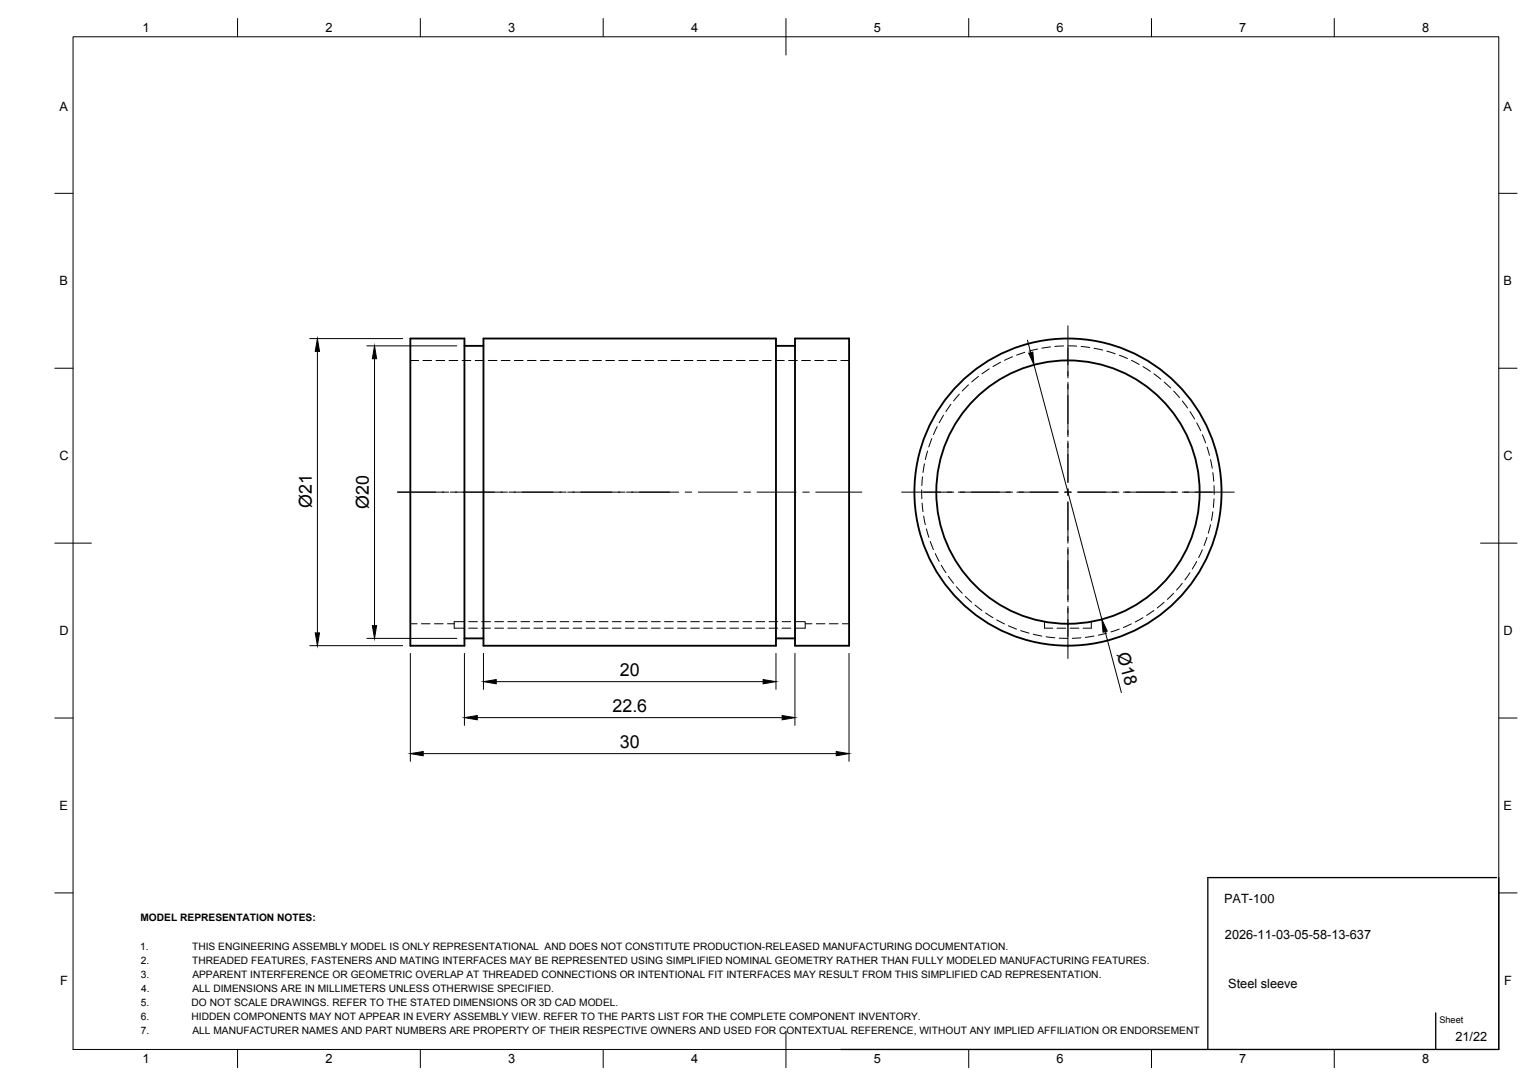
ISO-10303-21;
HEADER;
/* Generated by software containing ST-Developer
 * from STEP Tools, Inc. (www.steptools.com) 
 */

FILE_DESCRIPTION(
/* description */ (''),
/* implementation_level */ '2;1');

FILE_NAME(
/* name */ 'Steel sleeve.step',
/* time_stamp */ '2026-10-29T16:43:51-07:00',
/* author */ (''),
/* organization */ (''),
/* preprocessor_version */ 'ST-DEVELOPER v20.2',
/* originating_system */ 'Autodesk Translation Framework v15.17.0.0',
/* authorisation */ '');

FILE_SCHEMA (('AUTOMOTIVE_DESIGN { 1 0 10303 214 3 1 1 }'));
ENDSEC;

DATA;
#10=MECHANICAL_DESIGN_GEOMETRIC_PRESENTATION_REPRESENTATION('',(#380),#10292);
#334=SHAPE_REPRESENTATION_RELATIONSHIP('SRR','None',#10432,#357);
#357=ADVANCED_BREP_SHAPE_REPRESENTATION('',(#401),#10284);
#380=STYLED_ITEM('',(#10642),#401);
#401=MANIFOLD_SOLID_BREP('Body1',#5024);
#501=FACE_BOUND('',#1291,.T.);
#502=FACE_BOUND('',#1294,.T.);
#503=FACE_BOUND('',#1297,.T.);
#504=FACE_BOUND('',#1300,.T.);
#505=FACE_BOUND('',#1303,.T.);
#506=FACE_BOUND('',#1306,.T.);
#507=FACE_BOUND('',#1308,.T.);
#650=PLANE('',#5633);
#651=PLANE('',#5635);
#652=PLANE('',#5636);
#653=PLANE('',#5638);
#654=PLANE('',#5639);
#655=PLANE('',#5640);
#656=PLANE('',#5645);
#657=PLANE('',#5649);
#658=PLANE('',#5653);
#659=PLANE('',#5657);
#660=PLANE('',#5661);
#902=FACE_OUTER_BOUND('',#1285,.T.);
#903=FACE_OUTER_BOUND('',#1286,.T.);
#904=FACE_OUTER_BOUND('',#1287,.T.);
#905=FACE_OUTER_BOUND('',#1288,.T.);
#906=FACE_OUTER_BOUND('',#1289,.T.);
#907=FACE_OUTER_BOUND('',#1290,.T.);
#908=FACE_OUTER_BOUND('',#1292,.T.);
#909=FACE_OUTER_BOUND('',#1293,.T.);
#910=FACE_OUTER_BOUND('',#1295,.T.);
#911=FACE_OUTER_BOUND('',#1296,.T.);
#912=FACE_OUTER_BOUND('',#1298,.T.);
#913=FACE_OUTER_BOUND('',#1299,.T.);
#914=FACE_OUTER_BOUND('',#1301,.T.);
#915=FACE_OUTER_BOUND('',#1302,.T.);
#916=FACE_OUTER_BOUND('',#1304,.T.);
#917=FACE_OUTER_BOUND('',#1305,.T.);
#918=FACE_OUTER_BOUND('',#1307,.T.);
#1285=EDGE_LOOP('',(#4265,#4266,#4267,#4268));
#1286=EDGE_LOOP('',(#4269,#4270,#4271,#4272));
#1287=EDGE_LOOP('',(#4273,#4274,#4275,#4276));
#1288=EDGE_LOOP('',(#4277,#4278,#4279,#4280));
#1289=EDGE_LOOP('',(#4281,#4282,#4283,#4284));
#1290=EDGE_LOOP('',(#4285));
#1291=EDGE_LOOP('',(#4286));
#1292=EDGE_LOOP('',(#4287,#4288,#4289,#4290));
#1293=EDGE_LOOP('',(#4291));
#1294=EDGE_LOOP('',(#4292));
#1295=EDGE_LOOP('',(#4293,#4294,#4295,#4296));
#1296=EDGE_LOOP('',(#4297));
#1297=EDGE_LOOP('',(#4298));
#1298=EDGE_LOOP('',(#4299,#4300,#4301,#4302));
#1299=EDGE_LOOP('',(#4303));
#1300=EDGE_LOOP('',(#4304));
#1301=EDGE_LOOP('',(#4305,#4306,#4307,#4308));
#1302=EDGE_LOOP('',(#4309));
#1303=EDGE_LOOP('',(#4310));
#1304=EDGE_LOOP('',(#4311,#4312,#4313,#4314));
#1305=EDGE_LOOP('',(#4315));
#1306=EDGE_LOOP('',(#4316));
#1307=EDGE_LOOP('',(#4317,#4318,#4319,#4320));
#1308=EDGE_LOOP('',(#4321,#4322,#4323,#4324));
#1683=LINE('',#9771,#2075);
#1684=LINE('',#9773,#2076);
#1685=LINE('',#9774,#2077);
#1686=LINE('',#9777,#2078);
#1687=LINE('',#9779,#2079);
#1688=LINE('',#9780,#2080);
#1689=LINE('',#9785,#2081);
#1690=LINE('',#9786,#2082);
#1691=LINE('',#9788,#2083);
#1692=LINE('',#9789,#2084);
#1693=LINE('',#9799,#2085);
#1694=LINE('',#9806,#2086);
#1695=LINE('',#9813,#2087);
#1696=LINE('',#9820,#2088);
#1697=LINE('',#9827,#2089);
#1698=LINE('',#9832,#2090);
#2075=VECTOR('',#6828,1.);
#2076=VECTOR('',#6829,1.);
#2077=VECTOR('',#6830,1.);
#2078=VECTOR('',#6833,1.);
#2079=VECTOR('',#6834,1.);
#2080=VECTOR('',#6835,1.);
#2081=VECTOR('',#6840,1.);
#2082=VECTOR('',#6841,1.);
#2083=VECTOR('',#6844,1.);
#2084=VECTOR('',#6845,1.);
#2085=VECTOR('',#6858,1.05);
#2086=VECTOR('',#6867,1.);
#2087=VECTOR('',#6876,1.05);
#2088=VECTOR('',#6885,1.);
#2089=VECTOR('',#6894,1.05);
#2090=VECTOR('',#6901,0.9);
#2328=CIRCLE('',#5634,0.9);
#2329=CIRCLE('',#5637,0.9);
#2330=CIRCLE('',#5641,1.05);
#2331=CIRCLE('',#5642,0.9);
#2332=CIRCLE('',#5644,1.05);
#2333=CIRCLE('',#5646,1.);
#2334=CIRCLE('',#5648,1.);
#2335=CIRCLE('',#5650,1.05);
#2336=CIRCLE('',#5652,1.05);
#2337=CIRCLE('',#5654,1.);
#2338=CIRCLE('',#5656,1.);
#2339=CIRCLE('',#5658,1.05);
#2340=CIRCLE('',#5660,1.05);
#2341=CIRCLE('',#5662,0.9);
#2675=VERTEX_POINT('',#9767);
#2676=VERTEX_POINT('',#9768);
#2677=VERTEX_POINT('',#9770);
#2678=VERTEX_POINT('',#9772);
#2679=VERTEX_POINT('',#9776);
#2680=VERTEX_POINT('',#9778);
#2681=VERTEX_POINT('',#9782);
#2682=VERTEX_POINT('',#9784);
#2683=VERTEX_POINT('',#9792);
#2684=VERTEX_POINT('',#9794);
#2685=VERTEX_POINT('',#9797);
#2686=VERTEX_POINT('',#9801);
#2687=VERTEX_POINT('',#9804);
#2688=VERTEX_POINT('',#9808);
#2689=VERTEX_POINT('',#9811);
#2690=VERTEX_POINT('',#9815);
#2691=VERTEX_POINT('',#9818);
#2692=VERTEX_POINT('',#9822);
#2693=VERTEX_POINT('',#9825);
#2694=VERTEX_POINT('',#9829);
#3223=EDGE_CURVE('',#2675,#2676,#2328,.T.);
#3224=EDGE_CURVE('',#2677,#2675,#1683,.T.);
#3225=EDGE_CURVE('',#2678,#2677,#1684,.T.);
#3226=EDGE_CURVE('',#2676,#2678,#1685,.T.);
#3227=EDGE_CURVE('',#2676,#2679,#1686,.T.);
#3228=EDGE_CURVE('',#2680,#2678,#1687,.T.);
#3229=EDGE_CURVE('',#2680,#2679,#1688,.T.);
#3230=EDGE_CURVE('',#2679,#2681,#2329,.T.);
#3231=EDGE_CURVE('',#2682,#2680,#1689,.T.);
#3232=EDGE_CURVE('',#2681,#2682,#1690,.T.);
#3233=EDGE_CURVE('',#2681,#2675,#1691,.T.);
#3234=EDGE_CURVE('',#2682,#2677,#1692,.T.);
#3235=EDGE_CURVE('',#2683,#2683,#2330,.T.);
#3236=EDGE_CURVE('',#2684,#2684,#2331,.T.);
#3237=EDGE_CURVE('',#2685,#2685,#2332,.T.);
#3238=EDGE_CURVE('',#2685,#2683,#1693,.T.);
#3239=EDGE_CURVE('',#2686,#2686,#2333,.T.);
#3240=EDGE_CURVE('',#2687,#2687,#2334,.T.);
#3241=EDGE_CURVE('',#2687,#2686,#1694,.T.);
#3242=EDGE_CURVE('',#2688,#2688,#2335,.T.);
#3243=EDGE_CURVE('',#2689,#2689,#2336,.T.);
#3244=EDGE_CURVE('',#2689,#2688,#1695,.T.);
#3245=EDGE_CURVE('',#2690,#2690,#2337,.T.);
#3246=EDGE_CURVE('',#2691,#2691,#2338,.T.);
#3247=EDGE_CURVE('',#2691,#2690,#1696,.T.);
#3248=EDGE_CURVE('',#2692,#2692,#2339,.T.);
#3249=EDGE_CURVE('',#2693,#2693,#2340,.T.);
#3250=EDGE_CURVE('',#2693,#2692,#1697,.T.);
#3251=EDGE_CURVE('',#2694,#2694,#2341,.T.);
#3252=EDGE_CURVE('',#2694,#2684,#1698,.T.);
#4265=ORIENTED_EDGE('',*,*,#3223,.F.);
#4266=ORIENTED_EDGE('',*,*,#3224,.F.);
#4267=ORIENTED_EDGE('',*,*,#3225,.F.);
#4268=ORIENTED_EDGE('',*,*,#3226,.F.);
#4269=ORIENTED_EDGE('',*,*,#3227,.F.);
#4270=ORIENTED_EDGE('',*,*,#3226,.T.);
#4271=ORIENTED_EDGE('',*,*,#3228,.F.);
#4272=ORIENTED_EDGE('',*,*,#3229,.T.);
#4273=ORIENTED_EDGE('',*,*,#3230,.F.);
#4274=ORIENTED_EDGE('',*,*,#3229,.F.);
#4275=ORIENTED_EDGE('',*,*,#3231,.F.);
#4276=ORIENTED_EDGE('',*,*,#3232,.F.);
#4277=ORIENTED_EDGE('',*,*,#3233,.F.);
#4278=ORIENTED_EDGE('',*,*,#3232,.T.);
#4279=ORIENTED_EDGE('',*,*,#3234,.T.);
#4280=ORIENTED_EDGE('',*,*,#3224,.T.);
#4281=ORIENTED_EDGE('',*,*,#3234,.F.);
#4282=ORIENTED_EDGE('',*,*,#3231,.T.);
#4283=ORIENTED_EDGE('',*,*,#3228,.T.);
#4284=ORIENTED_EDGE('',*,*,#3225,.T.);
#4285=ORIENTED_EDGE('',*,*,#3235,.F.);
#4286=ORIENTED_EDGE('',*,*,#3236,.T.);
#4287=ORIENTED_EDGE('',*,*,#3237,.F.);
#4288=ORIENTED_EDGE('',*,*,#3238,.T.);
#4289=ORIENTED_EDGE('',*,*,#3235,.T.);
#4290=ORIENTED_EDGE('',*,*,#3238,.F.);
#4291=ORIENTED_EDGE('',*,*,#3237,.T.);
#4292=ORIENTED_EDGE('',*,*,#3239,.F.);
#4293=ORIENTED_EDGE('',*,*,#3240,.F.);
#4294=ORIENTED_EDGE('',*,*,#3241,.T.);
#4295=ORIENTED_EDGE('',*,*,#3239,.T.);
#4296=ORIENTED_EDGE('',*,*,#3241,.F.);
#4297=ORIENTED_EDGE('',*,*,#3242,.F.);
#4298=ORIENTED_EDGE('',*,*,#3240,.T.);
#4299=ORIENTED_EDGE('',*,*,#3243,.F.);
#4300=ORIENTED_EDGE('',*,*,#3244,.T.);
#4301=ORIENTED_EDGE('',*,*,#3242,.T.);
#4302=ORIENTED_EDGE('',*,*,#3244,.F.);
#4303=ORIENTED_EDGE('',*,*,#3243,.T.);
#4304=ORIENTED_EDGE('',*,*,#3245,.F.);
#4305=ORIENTED_EDGE('',*,*,#3246,.F.);
#4306=ORIENTED_EDGE('',*,*,#3247,.T.);
#4307=ORIENTED_EDGE('',*,*,#3245,.T.);
#4308=ORIENTED_EDGE('',*,*,#3247,.F.);
#4309=ORIENTED_EDGE('',*,*,#3248,.F.);
#4310=ORIENTED_EDGE('',*,*,#3246,.T.);
#4311=ORIENTED_EDGE('',*,*,#3249,.F.);
#4312=ORIENTED_EDGE('',*,*,#3250,.T.);
#4313=ORIENTED_EDGE('',*,*,#3248,.T.);
#4314=ORIENTED_EDGE('',*,*,#3250,.F.);
#4315=ORIENTED_EDGE('',*,*,#3249,.T.);
#4316=ORIENTED_EDGE('',*,*,#3251,.F.);
#4317=ORIENTED_EDGE('',*,*,#3251,.T.);
#4318=ORIENTED_EDGE('',*,*,#3252,.T.);
#4319=ORIENTED_EDGE('',*,*,#3236,.F.);
#4320=ORIENTED_EDGE('',*,*,#3252,.F.);
#4321=ORIENTED_EDGE('',*,*,#3230,.T.);
#4322=ORIENTED_EDGE('',*,*,#3233,.T.);
#4323=ORIENTED_EDGE('',*,*,#3223,.T.);
#4324=ORIENTED_EDGE('',*,*,#3227,.T.);
#4695=CYLINDRICAL_SURFACE('',#5643,1.05);
#4696=CYLINDRICAL_SURFACE('',#5647,1.);
#4697=CYLINDRICAL_SURFACE('',#5651,1.05);
#4698=CYLINDRICAL_SURFACE('',#5655,1.);
#4699=CYLINDRICAL_SURFACE('',#5659,1.05);
#4700=CYLINDRICAL_SURFACE('',#5663,0.9);
#4911=ADVANCED_FACE('',(#902),#650,.F.);
#4912=ADVANCED_FACE('',(#903),#651,.F.);
#4913=ADVANCED_FACE('',(#904),#652,.F.);
#4914=ADVANCED_FACE('',(#905),#653,.F.);
#4915=ADVANCED_FACE('',(#906),#654,.F.);
#4916=ADVANCED_FACE('',(#907,#501),#655,.T.);
#4917=ADVANCED_FACE('',(#908),#4695,.T.);
#4918=ADVANCED_FACE('',(#909,#502),#656,.T.);
#4919=ADVANCED_FACE('',(#910),#4696,.T.);
#4920=ADVANCED_FACE('',(#911,#503),#657,.T.);
#4921=ADVANCED_FACE('',(#912),#4697,.T.);
#4922=ADVANCED_FACE('',(#913,#504),#658,.T.);
#4923=ADVANCED_FACE('',(#914),#4698,.T.);
#4924=ADVANCED_FACE('',(#915,#505),#659,.T.);
#4925=ADVANCED_FACE('',(#916),#4699,.T.);
#4926=ADVANCED_FACE('',(#917,#506),#660,.T.);
#4927=ADVANCED_FACE('',(#918,#507),#4700,.F.);
#5024=CLOSED_SHELL('',(#4911,#4912,#4913,#4914,#4915,#4916,#4917,#4918,
#4919,#4920,#4921,#4922,#4923,#4924,#4925,#4926,#4927));
#5632=AXIS2_PLACEMENT_3D('',#9765,#6822,#6823);
#5633=AXIS2_PLACEMENT_3D('',#9766,#6824,#6825);
#5634=AXIS2_PLACEMENT_3D('',#9769,#6826,#6827);
#5635=AXIS2_PLACEMENT_3D('',#9775,#6831,#6832);
#5636=AXIS2_PLACEMENT_3D('',#9781,#6836,#6837);
#5637=AXIS2_PLACEMENT_3D('',#9783,#6838,#6839);
#5638=AXIS2_PLACEMENT_3D('',#9787,#6842,#6843);
#5639=AXIS2_PLACEMENT_3D('',#9790,#6846,#6847);
#5640=AXIS2_PLACEMENT_3D('',#9791,#6848,#6849);
#5641=AXIS2_PLACEMENT_3D('',#9793,#6850,#6851);
#5642=AXIS2_PLACEMENT_3D('',#9795,#6852,#6853);
#5643=AXIS2_PLACEMENT_3D('',#9796,#6854,#6855);
#5644=AXIS2_PLACEMENT_3D('',#9798,#6856,#6857);
#5645=AXIS2_PLACEMENT_3D('',#9800,#6859,#6860);
#5646=AXIS2_PLACEMENT_3D('',#9802,#6861,#6862);
#5647=AXIS2_PLACEMENT_3D('',#9803,#6863,#6864);
#5648=AXIS2_PLACEMENT_3D('',#9805,#6865,#6866);
#5649=AXIS2_PLACEMENT_3D('',#9807,#6868,#6869);
#5650=AXIS2_PLACEMENT_3D('',#9809,#6870,#6871);
#5651=AXIS2_PLACEMENT_3D('',#9810,#6872,#6873);
#5652=AXIS2_PLACEMENT_3D('',#9812,#6874,#6875);
#5653=AXIS2_PLACEMENT_3D('',#9814,#6877,#6878);
#5654=AXIS2_PLACEMENT_3D('',#9816,#6879,#6880);
#5655=AXIS2_PLACEMENT_3D('',#9817,#6881,#6882);
#5656=AXIS2_PLACEMENT_3D('',#9819,#6883,#6884);
#5657=AXIS2_PLACEMENT_3D('',#9821,#6886,#6887);
#5658=AXIS2_PLACEMENT_3D('',#9823,#6888,#6889);
#5659=AXIS2_PLACEMENT_3D('',#9824,#6890,#6891);
#5660=AXIS2_PLACEMENT_3D('',#9826,#6892,#6893);
#5661=AXIS2_PLACEMENT_3D('',#9828,#6895,#6896);
#5662=AXIS2_PLACEMENT_3D('',#9830,#6897,#6898);
#5663=AXIS2_PLACEMENT_3D('',#9831,#6899,#6900);
#6822=DIRECTION('axis',(0.,0.,1.));
#6823=DIRECTION('refdir',(1.,0.,0.));
#6824=DIRECTION('center_axis',(0.,1.,0.));
#6825=DIRECTION('ref_axis',(0.,0.,1.));
#6826=DIRECTION('center_axis',(0.,-1.,0.));
#6827=DIRECTION('ref_axis',(1.,0.,0.));
#6828=DIRECTION('',(-1.,0.,0.));
#6829=DIRECTION('',(0.,0.,-1.));
#6830=DIRECTION('',(1.,0.,0.));
#6831=DIRECTION('center_axis',(0.,0.,1.));
#6832=DIRECTION('ref_axis',(1.,0.,0.));
#6833=DIRECTION('',(0.,-1.,0.));
#6834=DIRECTION('',(0.,1.,0.));
#6835=DIRECTION('',(-1.,0.,0.));
#6836=DIRECTION('center_axis',(0.,-1.,0.));
#6837=DIRECTION('ref_axis',(0.,0.,-1.));
#6838=DIRECTION('center_axis',(0.,1.,0.));
#6839=DIRECTION('ref_axis',(1.,0.,0.));
#6840=DIRECTION('',(0.,0.,1.));
#6841=DIRECTION('',(1.,0.,0.));
#6842=DIRECTION('center_axis',(0.,0.,-1.));
#6843=DIRECTION('ref_axis',(-1.,0.,0.));
#6844=DIRECTION('',(0.,1.,0.));
#6845=DIRECTION('',(0.,1.,0.));
#6846=DIRECTION('center_axis',(1.,0.,0.));
#6847=DIRECTION('ref_axis',(0.,0.,-1.));
#6848=DIRECTION('center_axis',(0.,1.,0.));
#6849=DIRECTION('ref_axis',(0.,0.,1.));
#6850=DIRECTION('center_axis',(0.,-1.,0.));
#6851=DIRECTION('ref_axis',(1.,0.,0.));
#6852=DIRECTION('center_axis',(0.,-1.,0.));
#6853=DIRECTION('ref_axis',(1.,0.,0.));
#6854=DIRECTION('center_axis',(0.,-1.,0.));
#6855=DIRECTION('ref_axis',(1.,0.,0.));
#6856=DIRECTION('center_axis',(0.,-1.,0.));
#6857=DIRECTION('ref_axis',(1.,0.,0.));
#6858=DIRECTION('',(0.,1.,0.));
#6859=DIRECTION('center_axis',(0.,-1.,0.));
#6860=DIRECTION('ref_axis',(0.,0.,-1.));
#6861=DIRECTION('center_axis',(0.,-1.,0.));
#6862=DIRECTION('ref_axis',(1.,0.,0.));
#6863=DIRECTION('center_axis',(0.,-1.,0.));
#6864=DIRECTION('ref_axis',(1.,0.,0.));
#6865=DIRECTION('center_axis',(0.,-1.,0.));
#6866=DIRECTION('ref_axis',(1.,0.,0.));
#6867=DIRECTION('',(0.,1.,0.));
#6868=DIRECTION('center_axis',(0.,1.,0.));
#6869=DIRECTION('ref_axis',(0.,0.,1.));
#6870=DIRECTION('center_axis',(0.,-1.,0.));
#6871=DIRECTION('ref_axis',(1.,0.,0.));
#6872=DIRECTION('center_axis',(0.,-1.,0.));
#6873=DIRECTION('ref_axis',(1.,0.,0.));
#6874=DIRECTION('center_axis',(0.,-1.,0.));
#6875=DIRECTION('ref_axis',(1.,0.,0.));
#6876=DIRECTION('',(0.,1.,0.));
#6877=DIRECTION('center_axis',(0.,-1.,0.));
#6878=DIRECTION('ref_axis',(0.,0.,-1.));
#6879=DIRECTION('center_axis',(0.,-1.,0.));
#6880=DIRECTION('ref_axis',(1.,0.,0.));
#6881=DIRECTION('center_axis',(0.,-1.,0.));
#6882=DIRECTION('ref_axis',(1.,0.,0.));
#6883=DIRECTION('center_axis',(0.,-1.,0.));
#6884=DIRECTION('ref_axis',(1.,0.,0.));
#6885=DIRECTION('',(0.,1.,0.));
#6886=DIRECTION('center_axis',(0.,1.,0.));
#6887=DIRECTION('ref_axis',(0.,0.,1.));
#6888=DIRECTION('center_axis',(0.,-1.,0.));
#6889=DIRECTION('ref_axis',(1.,0.,0.));
#6890=DIRECTION('center_axis',(0.,-1.,0.));
#6891=DIRECTION('ref_axis',(1.,0.,0.));
#6892=DIRECTION('center_axis',(0.,-1.,0.));
#6893=DIRECTION('ref_axis',(1.,0.,0.));
#6894=DIRECTION('',(0.,1.,0.));
#6895=DIRECTION('center_axis',(0.,-1.,0.));
#6896=DIRECTION('ref_axis',(0.,0.,-1.));
#6897=DIRECTION('center_axis',(0.,-1.,0.));
#6898=DIRECTION('ref_axis',(1.,0.,0.));
#6899=DIRECTION('center_axis',(0.,-1.,0.));
#6900=DIRECTION('ref_axis',(1.,0.,0.));
#6901=DIRECTION('',(0.,1.,0.));
#9765=CARTESIAN_POINT('',(0.,0.,0.));
#9766=CARTESIAN_POINT('Origin',(0.75,1.2,0.));
#9767=CARTESIAN_POINT('',(0.885663593019381,1.2,-0.16));
#9768=CARTESIAN_POINT('',(0.885663593019381,1.2,0.16));
#9769=CARTESIAN_POINT('Origin',(0.,1.2,0.));
#9770=CARTESIAN_POINT('',(0.93,1.2,-0.16));
#9771=CARTESIAN_POINT('',(0.93,1.2,-0.16));
#9772=CARTESIAN_POINT('',(0.93,1.2,0.16));
#9773=CARTESIAN_POINT('',(0.93,1.2,0.16));
#9774=CARTESIAN_POINT('',(0.57,1.2,0.16));
#9775=CARTESIAN_POINT('Origin',(0.57,0.,0.16));
#9776=CARTESIAN_POINT('',(0.885663593019381,-1.2,0.16));
#9777=CARTESIAN_POINT('',(0.885663593019381,0.,0.16));
#9778=CARTESIAN_POINT('',(0.93,-1.2,0.16));
#9779=CARTESIAN_POINT('',(0.93,0.,0.16));
#9780=CARTESIAN_POINT('',(0.57,-1.2,0.16));
#9781=CARTESIAN_POINT('Origin',(0.75,-1.2,0.));
#9782=CARTESIAN_POINT('',(0.885663593019381,-1.2,-0.16));
#9783=CARTESIAN_POINT('Origin',(0.,-1.2,0.));
#9784=CARTESIAN_POINT('',(0.93,-1.2,-0.16));
#9785=CARTESIAN_POINT('',(0.93,-1.2,0.16));
#9786=CARTESIAN_POINT('',(0.93,-1.2,-0.16));
#9787=CARTESIAN_POINT('Origin',(0.93,0.,-0.16));
#9788=CARTESIAN_POINT('',(0.885663593019381,0.,-0.16));
#9789=CARTESIAN_POINT('',(0.93,0.,-0.16));
#9790=CARTESIAN_POINT('Origin',(0.93,0.,0.16));
#9791=CARTESIAN_POINT('Origin',(1.05,1.5,0.));
#9792=CARTESIAN_POINT('',(-1.05,1.5,-1.28587913910472E-16));
#9793=CARTESIAN_POINT('Origin',(0.,1.5,0.));
#9794=CARTESIAN_POINT('',(-0.9,1.5,-1.10218211923262E-16));
#9795=CARTESIAN_POINT('Origin',(0.,1.5,0.));
#9796=CARTESIAN_POINT('Origin',(0.,1.315,0.));
#9797=CARTESIAN_POINT('',(-1.05,1.13,-1.28587913910472E-16));
#9798=CARTESIAN_POINT('Origin',(0.,1.13,0.));
#9799=CARTESIAN_POINT('',(-1.05,1.315,-1.28587913910472E-16));
#9800=CARTESIAN_POINT('Origin',(1.,1.13,0.));
#9801=CARTESIAN_POINT('',(-1.,1.13,-1.22464679914735E-16));
#9802=CARTESIAN_POINT('Origin',(0.,1.13,0.));
#9803=CARTESIAN_POINT('Origin',(0.,1.065,0.));
#9804=CARTESIAN_POINT('',(-1.,1.,-1.22464679914735E-16));
#9805=CARTESIAN_POINT('Origin',(0.,1.,0.));
#9806=CARTESIAN_POINT('',(-1.,1.065,-1.22464679914735E-16));
#9807=CARTESIAN_POINT('Origin',(1.05,1.,0.));
#9808=CARTESIAN_POINT('',(-1.05,1.,-1.28587913910472E-16));
#9809=CARTESIAN_POINT('Origin',(0.,1.,0.));
#9810=CARTESIAN_POINT('Origin',(0.,0.,0.));
#9811=CARTESIAN_POINT('',(-1.05,-1.,-1.28587913910472E-16));
#9812=CARTESIAN_POINT('Origin',(0.,-1.,0.));
#9813=CARTESIAN_POINT('',(-1.05,0.,-1.28587913910472E-16));
#9814=CARTESIAN_POINT('Origin',(1.,-1.,0.));
#9815=CARTESIAN_POINT('',(-1.,-1.,-1.22464679914735E-16));
#9816=CARTESIAN_POINT('Origin',(0.,-1.,0.));
#9817=CARTESIAN_POINT('Origin',(0.,-1.065,0.));
#9818=CARTESIAN_POINT('',(-1.,-1.13,-1.22464679914735E-16));
#9819=CARTESIAN_POINT('Origin',(0.,-1.13,0.));
#9820=CARTESIAN_POINT('',(-1.,-1.065,-1.22464679914735E-16));
#9821=CARTESIAN_POINT('Origin',(1.05,-1.13,0.));
#9822=CARTESIAN_POINT('',(-1.05,-1.13,-1.28587913910472E-16));
#9823=CARTESIAN_POINT('Origin',(0.,-1.13,0.));
#9824=CARTESIAN_POINT('Origin',(0.,-1.315,0.));
#9825=CARTESIAN_POINT('',(-1.05,-1.5,-1.28587913910472E-16));
#9826=CARTESIAN_POINT('Origin',(0.,-1.5,0.));
#9827=CARTESIAN_POINT('',(-1.05,-1.315,-1.28587913910472E-16));
#9828=CARTESIAN_POINT('Origin',(0.9,-1.5,0.));
#9829=CARTESIAN_POINT('',(-0.9,-1.5,-1.10218211923262E-16));
#9830=CARTESIAN_POINT('Origin',(0.,-1.5,0.));
#9831=CARTESIAN_POINT('Origin',(0.,0.,0.));
#9832=CARTESIAN_POINT('',(-0.9,0.,-1.10218211923262E-16));
#10256=UNCERTAINTY_MEASURE_WITH_UNIT(LENGTH_MEASURE(0.001),#10293,
'DISTANCE_ACCURACY_VALUE',
'Maximum model space distance between geometric entities at asserted c
onnectivities');
#10264=UNCERTAINTY_MEASURE_WITH_UNIT(LENGTH_MEASURE(0.001),#10293,
'DISTANCE_ACCURACY_VALUE',
'Maximum model space distance between geometric entities at asserted c
onnectivities');
#10284=(
GEOMETRIC_REPRESENTATION_CONTEXT(3)
GLOBAL_UNCERTAINTY_ASSIGNED_CONTEXT((#10256))
GLOBAL_UNIT_ASSIGNED_CONTEXT((#10293,#10295,#10296))
REPRESENTATION_CONTEXT('','3D')
);
#10292=(
GEOMETRIC_REPRESENTATION_CONTEXT(3)
GLOBAL_UNCERTAINTY_ASSIGNED_CONTEXT((#10264))
GLOBAL_UNIT_ASSIGNED_CONTEXT((#10293,#10295,#10296))
REPRESENTATION_CONTEXT('','3D')
);
#10293=(
LENGTH_UNIT()
NAMED_UNIT(*)
SI_UNIT(.CENTI.,.METRE.)
);
#10295=(
NAMED_UNIT(*)
PLANE_ANGLE_UNIT()
SI_UNIT($,.RADIAN.)
);
#10296=(
NAMED_UNIT(*)
SI_UNIT($,.STERADIAN.)
SOLID_ANGLE_UNIT()
);
#10316=SHAPE_DEFINITION_REPRESENTATION(#10343,#10432);
#10343=PRODUCT_DEFINITION_SHAPE('',$,#10460);
#10432=SHAPE_REPRESENTATION('',(#5632),#10284);
#10440=PRODUCT_DEFINITION_CONTEXT('part definition',#10523,'design');
#10460=PRODUCT_DEFINITION('Steel sleeve','Steel sleeve',#10487,
#10440);
#10487=PRODUCT_DEFINITION_FORMATION('',$,#10544);
#10523=APPLICATION_CONTEXT(
'Core Data for Automotive Mechanical Design Process');
#10524=PRODUCT_CONTEXT('part definition',#10523,'mechanical');
#10544=PRODUCT('Steel sleeve','Steel sleeve','Steel sleeve',
(#10524));
#10636=COLOUR_RGB('Off White',0.89,0.88,0.83);
#10637=FILL_AREA_STYLE_COLOUR('',#10636);
#10638=FILL_AREA_STYLE('',(#10637));
#10639=SURFACE_STYLE_FILL_AREA(#10638);
#10640=SURFACE_SIDE_STYLE('',(#10639));
#10641=SURFACE_STYLE_USAGE(.BOTH.,#10640);
#10642=PRESENTATION_STYLE_ASSIGNMENT((#10641));
ENDSEC;
END-ISO-10303-21;
